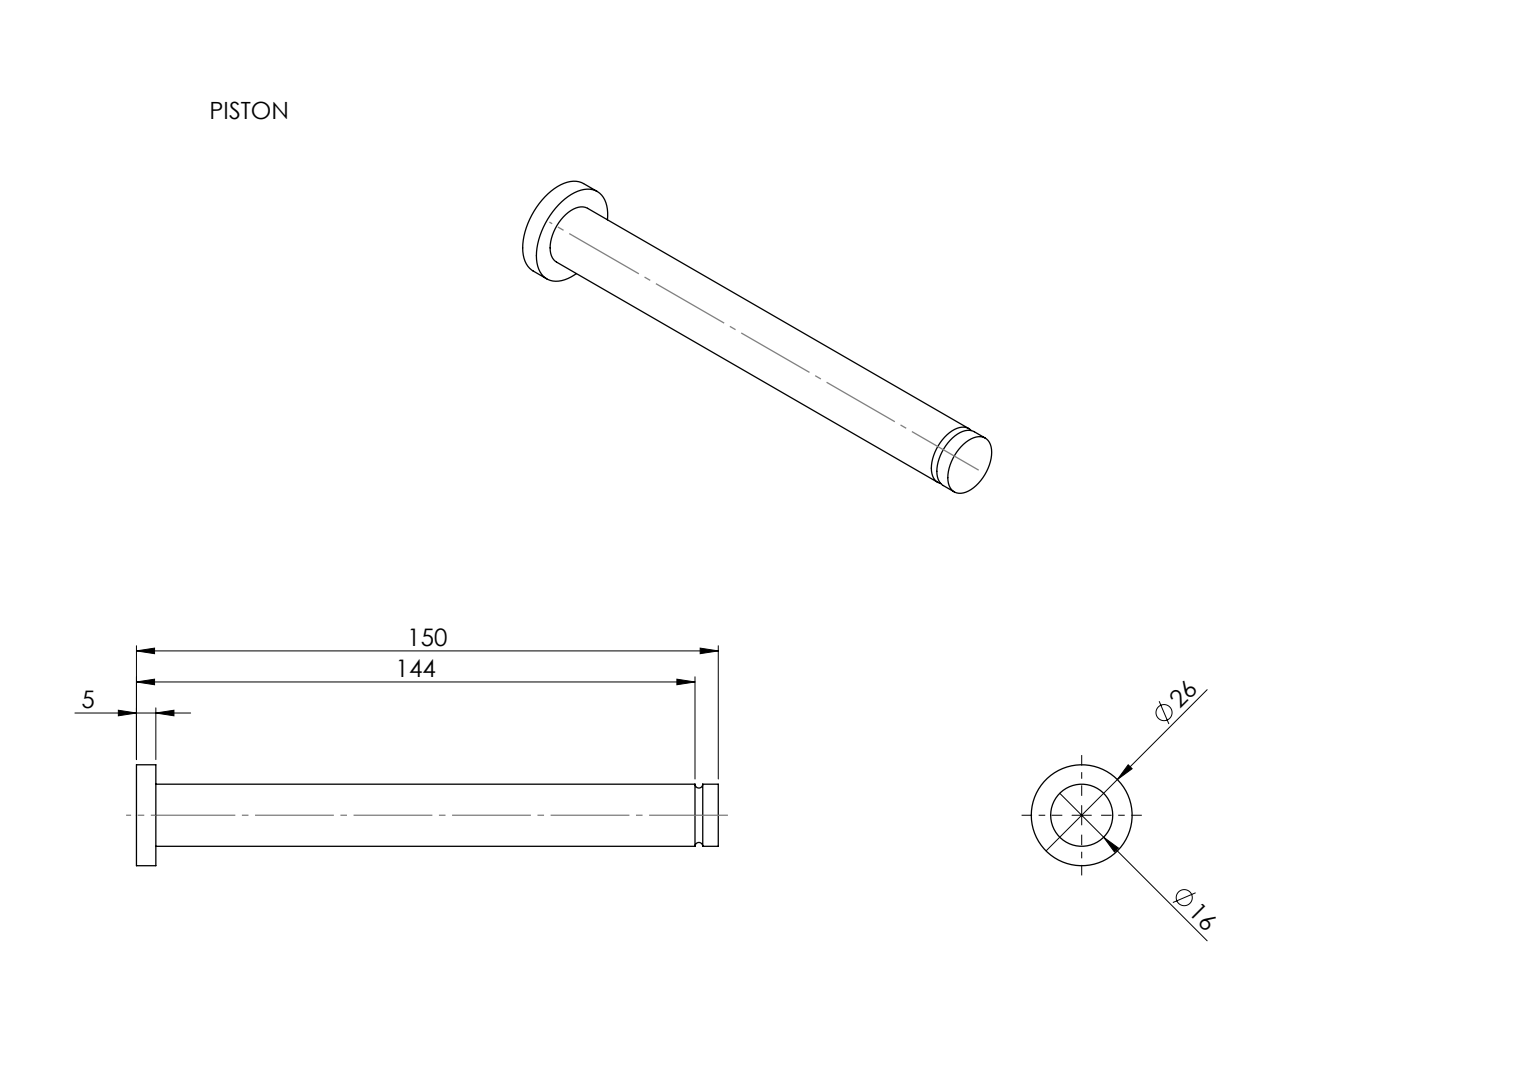
ISO-10303-21;
HEADER;
FILE_DESCRIPTION (('STEP AP214'),
    '1' );
FILE_NAME ('piston.step',
    '2026-10-08T13:22:57',
    ( '' ),
    ( '' ),
    'SwSTEP 2.0',
    'SolidWorks 2026',
    '' );
FILE_SCHEMA (( 'AUTOMOTIVE_DESIGN' ));
ENDSEC;

DATA;
#18=AXIS2_PLACEMENT_3D ( 'NONE', #9607, #4018, #5606 ) ;
#52=CIRCLE ( 'NONE', #2688, 13.00000000000000000 ) ;
#70=DIRECTION ( 'NONE',  ( 0.000000000000000000, 0.000000000000000000, 1.000000000000000000 ) ) ;
#115=ORIENTED_EDGE ( 'NONE', *, *, #1311, .F. ) ;
#116=STYLED_ITEM ( 'NONE', ( #9052 ), #3700 ) ;
#154=ORIENTED_EDGE ( 'NONE', *, *, #7460, .T. ) ;
#166=VERTEX_POINT ( 'NONE', #3235 ) ;
#178=ADVANCED_FACE ( 'NONE', ( #1639 ), #6426, .T. ) ;
#212=DIRECTION ( 'NONE',  ( 0.000000000000000000, -1.224646799147353454E-16, 1.000000000000000000 ) ) ;
#224=LINE ( 'NONE', #5694, #1710 ) ;
#245=CARTESIAN_POINT ( 'NONE',  ( 0.000000000000000000, 0.000000000000000000, 0.000000000000000000 ) ) ;
#252=ORIENTED_EDGE ( 'NONE', *, *, #5467, .F. ) ;
#395=CARTESIAN_POINT ( 'NONE',  ( 56.99999999999997158, 0.000000000000000000, 0.000000000000000000 ) ) ;
#422=DIRECTION ( 'NONE',  ( -1.000000000000000000, -0.000000000000000000, -0.000000000000000000 ) ) ;
#457=EDGE_CURVE ( 'NONE', #4209, #166, #5446, .T. ) ;
#458=ORIENTED_EDGE ( 'NONE', *, *, #1070, .T. ) ;
#467=EDGE_LOOP ( 'NONE', ( #5213, #7257 ) ) ;
#481=DIRECTION ( 'NONE',  ( 0.000000000000000000, -1.000000000000000000, 0.000000000000000000 ) ) ;
#568=ADVANCED_BREP_SHAPE_REPRESENTATION ( '', ( #3700, #3995 ), #9548 ) ;
#570=AXIS2_PLACEMENT_3D ( 'NONE', #1238, #4444, #4391 ) ;
#580=SHAPE_REPRESENTATION_RELATIONSHIP ( 'NONE' , 'NONE' ,  #8907, #568 ) ;
#635=COLOUR_RGB ( '', 0.09019608, 0.27058824, 0.51372549) ;
#653=DIRECTION ( 'NONE',  ( -1.000000000000000000, 0.000000000000000000, -0.000000000000000000 ) ) ;
#661=DIRECTION ( 'NONE',  ( -1.000000000000000000, -0.000000000000000000, -0.000000000000000000 ) ) ;
#689=AXIS2_PLACEMENT_3D ( 'NONE', #1610, #4761, #212 ) ;
#704=CYLINDRICAL_SURFACE ( 'NONE', #8270, 8.000000000000000000 ) ;
#754=DIRECTION ( 'NONE',  ( -1.000000000000000000, -0.000000000000000000, -0.000000000000000000 ) ) ;
#784=ORIENTED_EDGE ( 'NONE', *, *, #8505, .T. ) ;
#788=CARTESIAN_POINT ( 'NONE',  ( 56.99999999999997158, 0.000000000000000000, 8.000000000000000000 ) ) ;
#813=UNCERTAINTY_MEASURE_WITH_UNIT (LENGTH_MEASURE( 1.000000000000000082E-05 ), #5110, 'distance_accuracy_value', 'NONE');
#844=FACE_OUTER_BOUND ( 'NONE', #5304, .T. ) ;
#928=VERTEX_POINT ( 'NONE', #4806 ) ;
#948=DIRECTION ( 'NONE',  ( -1.000000000000000000, -0.000000000000000000, -0.000000000000000000 ) ) ;
#980=ORIENTED_EDGE ( 'NONE', *, *, #1070, .F. ) ;
#1002=CARTESIAN_POINT ( 'NONE',  ( 56.99999999999997158, 0.000000000000000000, 0.000000000000000000 ) ) ;
#1027=TOROIDAL_SURFACE ( 'NONE', #1374, 8.000000000000000000, 1.000000000000000888 ) ;
#1037=ADVANCED_FACE ( 'NONE', ( #8531 ), #4657, .T. ) ;
#1059=CARTESIAN_POINT ( 'NONE',  ( 56.99999999999997158, 0.000000000000000000, 0.000000000000000000 ) ) ;
#1068=CIRCLE ( 'NONE', #6816, 8.000000000000000000 ) ;
#1070=EDGE_CURVE ( 'NONE', #9896, #4112, #1160, .T. ) ;
#1101=SURFACE_STYLE_USAGE ( .BOTH. , #1873 ) ;
#1108=CARTESIAN_POINT ( 'NONE',  ( -83.00000000000001421, 0.000000000000000000, 0.000000000000000000 ) ) ;
#1160=CIRCLE ( 'NONE', #5118, 1.000000000000000888 ) ;
#1238=CARTESIAN_POINT ( 'NONE',  ( -88.00000000000002842, 0.000000000000000000, 0.000000000000000000 ) ) ;
#1311=EDGE_CURVE ( 'NONE', #9896, #7728, #8253, .T. ) ;
#1317=DIRECTION ( 'NONE',  ( 0.000000000000000000, 0.000000000000000000, 1.000000000000000000 ) ) ;
#1370=CARTESIAN_POINT ( 'NONE',  ( -88.00000000000002842, 0.000000000000000000, 0.000000000000000000 ) ) ;
#1374=AXIS2_PLACEMENT_3D ( 'NONE', #1059, #5794, #8174 ) ;
#1408=CARTESIAN_POINT ( 'NONE',  ( -88.00000000000002842, 0.000000000000000000, 8.000000000000000000 ) ) ;
#1416=DIRECTION ( 'NONE',  ( -1.000000000000000000, -0.000000000000000000, -0.000000000000000000 ) ) ;
#1423=EDGE_LOOP ( 'NONE', ( #9348, #2777, #5681, #2103 ) ) ;
#1425=DIRECTION ( 'NONE',  ( 0.000000000000000000, 0.000000000000000000, 1.000000000000000000 ) ) ;
#1482=CARTESIAN_POINT ( 'NONE',  ( 56.99999999999997158, 0.000000000000000000, 6.999999999999999112 ) ) ;
#1486=CARTESIAN_POINT ( 'NONE',  ( 57.99999999999997158, 0.000000000000000000, 8.000000000000000000 ) ) ;
#1526=AXIS2_PLACEMENT_3D ( 'NONE', #4077, #8682, #4034 ) ;
#1553=ORIENTED_EDGE ( 'NONE', *, *, #2011, .T. ) ;
#1569=DIRECTION ( 'NONE',  ( 0.000000000000000000, 0.000000000000000000, -1.000000000000000000 ) ) ;
#1589=DIRECTION ( 'NONE',  ( -1.000000000000000000, -0.000000000000000000, -0.000000000000000000 ) ) ;
#1610=CARTESIAN_POINT ( 'NONE',  ( 56.99999999999997158, 9.797174393178825657E-16, -8.000000000000000000 ) ) ;
#1639=FACE_OUTER_BOUND ( 'NONE', #6518, .T. ) ;
#1662=AXIS2_PLACEMENT_3D ( 'NONE', #3535, #4306, #3624 ) ;
#1692=VERTEX_POINT ( 'NONE', #7477 ) ;
#1705=VERTEX_POINT ( 'NONE', #2871 ) ;
#1710=VECTOR ( 'NONE', #8816, 1000.000000000000000 ) ;
#1810=VERTEX_POINT ( 'NONE', #1486 ) ;
#1822=DIRECTION ( 'NONE',  ( -1.000000000000000000, -0.000000000000000000, -0.000000000000000000 ) ) ;
#1833=CIRCLE ( 'NONE', #2488, 8.000000000000000000 ) ;
#1864=DIRECTION ( 'NONE',  ( -1.000000000000000000, -0.000000000000000000, -0.000000000000000000 ) ) ;
#1873=SURFACE_SIDE_STYLE ('',( #8961 ) ) ;
#1913=SURFACE_SIDE_STYLE ('',( #7386 ) ) ;
#1914=CARTESIAN_POINT ( 'NONE',  ( 55.99999999999996447, 0.000000000000000000, 0.000000000000000000 ) ) ;
#1984=DIRECTION ( 'NONE',  ( -1.000000000000000000, -0.000000000000000000, -0.000000000000000000 ) ) ;
#1985=CIRCLE ( 'NONE', #2326, 8.000000000000000000 ) ;
#2011=EDGE_CURVE ( 'NONE', #1692, #2905, #7742, .T. ) ;
#2027=CARTESIAN_POINT ( 'NONE',  ( 56.99999999999997158, 0.000000000000000000, 8.000000000000000000 ) ) ;
#2033=DIRECTION ( 'NONE',  ( 0.000000000000000000, 0.000000000000000000, 1.000000000000000000 ) ) ;
#2054=ORIENTED_EDGE ( 'NONE', *, *, #3567, .F. ) ;
#2061=EDGE_LOOP ( 'NONE', ( #252, #784, #3897, #9819 ) ) ;
#2103=ORIENTED_EDGE ( 'NONE', *, *, #6989, .F. ) ;
#2126=EDGE_CURVE ( 'NONE', #9861, #928, #5621, .T. ) ;
#2163=CIRCLE ( 'NONE', #3319, 6.999999999999999112 ) ;
#2196=ORIENTED_EDGE ( 'NONE', *, *, #2684, .F. ) ;
#2248=DIRECTION ( 'NONE',  ( -0.000000000000000000, 0.000000000000000000, 1.000000000000000000 ) ) ;
#2269=ORIENTED_EDGE ( 'NONE', *, *, #5485, .T. ) ;
#2326=AXIS2_PLACEMENT_3D ( 'NONE', #4570, #9220, #7774 ) ;
#2380=AXIS2_PLACEMENT_3D ( 'NONE', #788, #4715, #1569 ) ;
#2390=CARTESIAN_POINT ( 'NONE',  ( -83.00000000000001421, 9.797174393178825657E-16, -8.000000000000000000 ) ) ;
#2395=FACE_OUTER_BOUND ( 'NONE', #1423, .T. ) ;
#2424=CARTESIAN_POINT ( 'NONE',  ( -83.00000000000001421, 0.000000000000000000, 13.00000000000000000 ) ) ;
#2488=AXIS2_PLACEMENT_3D ( 'NONE', #8057, #7287, #3931 ) ;
#2535=EDGE_CURVE ( 'NONE', #2905, #166, #5283, .T. ) ;
#2550=DIRECTION ( 'NONE',  ( 0.000000000000000000, 0.000000000000000000, 1.000000000000000000 ) ) ;
#2591=DIRECTION ( 'NONE',  ( 0.000000000000000000, 0.000000000000000000, 1.000000000000000000 ) ) ;
#2597=DIRECTION ( 'NONE',  ( 0.000000000000000000, 0.000000000000000000, 1.000000000000000000 ) ) ;
#2611=PRODUCT_DEFINITION_FORMATION_WITH_SPECIFIED_SOURCE ( 'ANY', '', #6639, .NOT_KNOWN. ) ;
#2682=CIRCLE ( 'NONE', #6305, 8.000000000000000000 ) ;
#2684=EDGE_CURVE ( 'NONE', #1705, #6462, #3540, .T. ) ;
#2688=AXIS2_PLACEMENT_3D ( 'NONE', #7784, #754, #70 ) ;
#2749=MECHANICAL_DESIGN_GEOMETRIC_PRESENTATION_REPRESENTATION('',(#116),#3578);
#2768=VERTEX_POINT ( 'NONE', #3014 ) ;
#2777=ORIENTED_EDGE ( 'NONE', *, *, #6679, .T. ) ;
#2800=ORIENTED_EDGE ( 'NONE', *, *, #4948, .F. ) ;
#2851=FACE_OUTER_BOUND ( 'NONE', #8992, .T. ) ;
#2860=PLANE ( 'NONE',  #9099 ) ;
#2869=ADVANCED_FACE ( 'NONE', ( #2395 ), #704, .T. ) ;
#2871=CARTESIAN_POINT ( 'NONE',  ( 55.99999999999996447, 0.000000000000000000, 8.000000000000000000 ) ) ;
#2905=VERTEX_POINT ( 'NONE', #9384 ) ;
#2973=ORIENTED_EDGE ( 'NONE', *, *, #8348, .T. ) ;
#2981=AXIS2_PLACEMENT_3D ( 'NONE', #7760, #6860, #10083 ) ;
#2991=ORIENTED_EDGE ( 'NONE', *, *, #457, .F. ) ;
#3014=CARTESIAN_POINT ( 'NONE',  ( 55.99999999999996447, 9.797174393178825657E-16, -8.000000000000000000 ) ) ;
#3018=CIRCLE ( 'NONE', #6628, 13.00000000000000000 ) ;
#3050=PLANE ( 'NONE',  #2981 ) ;
#3089=COLOUR_RGB ( '', 0.09019608, 0.27058824, 0.51372549) ;
#3099=DIRECTION ( 'NONE',  ( 0.000000000000000000, 0.000000000000000000, 1.000000000000000000 ) ) ;
#3101=DIRECTION ( 'NONE',  ( -1.000000000000000000, -0.000000000000000000, -0.000000000000000000 ) ) ;
#3146=CIRCLE ( 'NONE', #5278, 8.000000000000000000 ) ;
#3183=EDGE_LOOP ( 'NONE', ( #115, #458, #8887, #6583 ) ) ;
#3210=AXIS2_PLACEMENT_3D ( 'NONE', #6299, #1416, #8541 ) ;
#3231=ORIENTED_EDGE ( 'NONE', *, *, #2126, .T. ) ;
#3235=CARTESIAN_POINT ( 'NONE',  ( -88.00000000000002842, 0.000000000000000000, 13.00000000000000000 ) ) ;
#3237=DIRECTION ( 'NONE',  ( -1.000000000000000000, -0.000000000000000000, -0.000000000000000000 ) ) ;
#3318=AXIS2_PLACEMENT_3D ( 'NONE', #1370, #9952, #2033 ) ;
#3319=AXIS2_PLACEMENT_3D ( 'NONE', #395, #8295, #5806 ) ;
#3353=ORIENTED_EDGE ( 'NONE', *, *, #1311, .T. ) ;
#3377=DIRECTION ( 'NONE',  ( -1.000000000000000000, -0.000000000000000000, -0.000000000000000000 ) ) ;
#3429=ORIENTED_EDGE ( 'NONE', *, *, #6679, .F. ) ;
#3494=PRODUCT_DEFINITION_CONTEXT ( 'detailed design', #4873, 'design' ) ;
#3535=CARTESIAN_POINT ( 'NONE',  ( -83.00000000000001421, 0.000000000000000000, 13.00000000000000000 ) ) ;
#3540=LINE ( 'NONE', #8290, #6746 ) ;
#3567=EDGE_CURVE ( 'NONE', #1705, #2768, #8869, .T. ) ;
#3578=( GEOMETRIC_REPRESENTATION_CONTEXT ( 3 ) GLOBAL_UNCERTAINTY_ASSIGNED_CONTEXT ( ( #813 ) ) GLOBAL_UNIT_ASSIGNED_CONTEXT ( ( #5110, #4336, #5926 ) ) REPRESENTATION_CONTEXT ( 'NONE', 'WORKASPACE' ) );
#3623=AXIS2_PLACEMENT_3D ( 'NONE', #3929, #7855, #3099 ) ;
#3624=DIRECTION ( 'NONE',  ( 0.000000000000000000, 0.000000000000000000, -1.000000000000000000 ) ) ;
#3660=CLOSED_SHELL ( 'NONE', ( #4316, #9400, #6703, #5314, #178, #6131, #7297, #8672, #8192, #2869, #5187, #1037, #9746 ) ) ;
#3669=EDGE_CURVE ( 'NONE', #2768, #9103, #8950, .T. ) ;
#3694=DIRECTION ( 'NONE',  ( -1.000000000000000000, -0.000000000000000000, -0.000000000000000000 ) ) ;
#3700=MANIFOLD_SOLID_BREP ( 'Revolve1', #3660 ) ;
#3706=ORIENTED_EDGE ( 'NONE', *, *, #2535, .F. ) ;
#3708=ORIENTED_EDGE ( 'NONE', *, *, #9778, .F. ) ;
#3874=ORIENTED_EDGE ( 'NONE', *, *, #10088, .T. ) ;
#3886=ORIENTED_EDGE ( 'NONE', *, *, #3567, .T. ) ;
#3897=ORIENTED_EDGE ( 'NONE', *, *, #9778, .T. ) ;
#3929=CARTESIAN_POINT ( 'NONE',  ( -88.00000000000002842, 0.000000000000000000, 0.000000000000000000 ) ) ;
#3931=DIRECTION ( 'NONE',  ( 0.000000000000000000, 0.000000000000000000, 1.000000000000000000 ) ) ;
#3958=ORIENTED_EDGE ( 'NONE', *, *, #5485, .F. ) ;
#3960=VECTOR ( 'NONE', #9493, 1000.000000000000000 ) ;
#3995=AXIS2_PLACEMENT_3D ( 'NONE', #245, #8930, #7419 ) ;
#3999=CYLINDRICAL_SURFACE ( 'NONE', #4635, 13.00000000000000000 ) ;
#4018=DIRECTION ( 'NONE',  ( -1.000000000000000000, -0.000000000000000000, -0.000000000000000000 ) ) ;
#4034=DIRECTION ( 'NONE',  ( 0.000000000000000000, 0.000000000000000000, 1.000000000000000000 ) ) ;
#4077=CARTESIAN_POINT ( 'NONE',  ( 56.99999999999997158, 0.000000000000000000, 0.000000000000000000 ) ) ;
#4110=DIRECTION ( 'NONE',  ( 0.000000000000000000, 0.000000000000000000, 1.000000000000000000 ) ) ;
#4112=VERTEX_POINT ( 'NONE', #6491 ) ;
#4209=VERTEX_POINT ( 'NONE', #2424 ) ;
#4233=FILL_AREA_STYLE ('',( #8159 ) ) ;
#4285=SURFACE_STYLE_USAGE ( .BOTH. , #1913 ) ;
#4306=DIRECTION ( 'NONE',  ( 1.000000000000000000, 0.000000000000000000, 0.000000000000000000 ) ) ;
#4316=ADVANCED_FACE ( 'NONE', ( #4802 ), #8796, .F. ) ;
#4336=( NAMED_UNIT ( * ) PLANE_ANGLE_UNIT ( ) SI_UNIT ( $, .RADIAN. ) );
#4360=EDGE_LOOP ( 'NONE', ( #3231, #5060, #5358, #3708 ) ) ;
#4391=DIRECTION ( 'NONE',  ( 0.000000000000000000, 0.000000000000000000, 1.000000000000000000 ) ) ;
#4444=DIRECTION ( 'NONE',  ( -1.000000000000000000, -0.000000000000000000, -0.000000000000000000 ) ) ;
#4570=CARTESIAN_POINT ( 'NONE',  ( 61.99999999999997158, 0.000000000000000000, 0.000000000000000000 ) ) ;
#4635=AXIS2_PLACEMENT_3D ( 'NONE', #9486, #948, #2591 ) ;
#4637=CARTESIAN_POINT ( 'NONE',  ( -88.00000000000002842, 1.592040838891559095E-15, -13.00000000000000000 ) ) ;
#4657=CYLINDRICAL_SURFACE ( 'NONE', #3623, 8.000000000000000000 ) ;
#4715=DIRECTION ( 'NONE',  ( 0.000000000000000000, -1.000000000000000000, 0.000000000000000000 ) ) ;
#4761=DIRECTION ( 'NONE',  ( -0.000000000000000000, 1.000000000000000000, 1.224646799147353207E-16 ) ) ;
#4800=AXIS2_PLACEMENT_3D ( 'NONE', #8667, #1589, #7108 ) ;
#4802=FACE_OUTER_BOUND ( 'NONE', #9503, .T. ) ;
#4806=CARTESIAN_POINT ( 'NONE',  ( 61.99999999999997158, 9.797174393178825657E-16, -8.000000000000000000 ) ) ;
#4873=APPLICATION_CONTEXT ( 'automotive_design' ) ;
#4891=DIRECTION ( 'NONE',  ( 0.000000000000000000, 0.000000000000000000, 1.000000000000000000 ) ) ;
#4948=EDGE_CURVE ( 'NONE', #166, #2905, #52, .T. ) ;
#4966=ORIENTED_EDGE ( 'NONE', *, *, #9912, .T. ) ;
#5012=ORIENTED_EDGE ( 'NONE', *, *, #7460, .F. ) ;
#5013=CARTESIAN_POINT ( 'NONE',  ( -88.00000000000002842, 9.797174393178825657E-16, -8.000000000000000000 ) ) ;
#5060=ORIENTED_EDGE ( 'NONE', *, *, #5467, .T. ) ;
#5062=DIRECTION ( 'NONE',  ( 0.000000000000000000, 0.000000000000000000, 1.000000000000000000 ) ) ;
#5089=FACE_OUTER_BOUND ( 'NONE', #467, .T. ) ;
#5110=( LENGTH_UNIT ( ) NAMED_UNIT ( * ) SI_UNIT ( .MILLI., .METRE. ) );
#5118=AXIS2_PLACEMENT_3D ( 'NONE', #9417, #7073, #9316 ) ;
#5120=( NAMED_UNIT ( * ) PLANE_ANGLE_UNIT ( ) SI_UNIT ( $, .RADIAN. ) );
#5131=VECTOR ( 'NONE', #3101, 1000.000000000000000 ) ;
#5177=PRODUCT_DEFINITION_SHAPE ( 'NONE', 'NONE',  #9415 ) ;
#5187=ADVANCED_FACE ( 'NONE', ( #9337 ), #1027, .F. ) ;
#5213=ORIENTED_EDGE ( 'NONE', *, *, #4948, .T. ) ;
#5278=AXIS2_PLACEMENT_3D ( 'NONE', #5584, #9533, #7243 ) ;
#5283=CIRCLE ( 'NONE', #3318, 13.00000000000000000 ) ;
#5304=EDGE_LOOP ( 'NONE', ( #7513, #2269, #8105, #3706 ) ) ;
#5314=ADVANCED_FACE ( 'NONE', ( #7302 ), #7146, .F. ) ;
#5328=LINE ( 'NONE', #1408, #5131 ) ;
#5330=PRESENTATION_STYLE_ASSIGNMENT (( #1101 ) ) ;
#5358=ORIENTED_EDGE ( 'NONE', *, *, #8807, .F. ) ;
#5360=ORIENTED_EDGE ( 'NONE', *, *, #7171, .F. ) ;
#5388=ORIENTED_EDGE ( 'NONE', *, *, #7171, .T. ) ;
#5408=( GEOMETRIC_REPRESENTATION_CONTEXT ( 3 ) GLOBAL_UNCERTAINTY_ASSIGNED_CONTEXT ( ( #9905 ) ) GLOBAL_UNIT_ASSIGNED_CONTEXT ( ( #5427, #5482, #7858 ) ) REPRESENTATION_CONTEXT ( 'NONE', 'WORKASPACE' ) );
#5427=( LENGTH_UNIT ( ) NAMED_UNIT ( * ) SI_UNIT ( .MILLI., .METRE. ) );
#5443=EDGE_CURVE ( 'NONE', #4112, #1810, #2682, .T. ) ;
#5446=LINE ( 'NONE', #8607, #3960 ) ;
#5467=EDGE_CURVE ( 'NONE', #928, #4112, #224, .T. ) ;
#5482=( NAMED_UNIT ( * ) PLANE_ANGLE_UNIT ( ) SI_UNIT ( $, .RADIAN. ) );
#5485=EDGE_CURVE ( 'NONE', #1692, #4209, #3018, .T. ) ;
#5584=CARTESIAN_POINT ( 'NONE',  ( 57.99999999999997158, 0.000000000000000000, 0.000000000000000000 ) ) ;
#5606=DIRECTION ( 'NONE',  ( 0.000000000000000000, 0.000000000000000000, 1.000000000000000000 ) ) ;
#5621=CIRCLE ( 'NONE', #4800, 8.000000000000000000 ) ;
#5681=ORIENTED_EDGE ( 'NONE', *, *, #2684, .T. ) ;
#5694=CARTESIAN_POINT ( 'NONE',  ( -88.00000000000002842, 9.797174393178825657E-16, -8.000000000000000000 ) ) ;
#5735=MECHANICAL_DESIGN_GEOMETRIC_PRESENTATION_REPRESENTATION('',(#7384),#5408);
#5740=DIRECTION ( 'NONE',  ( -1.000000000000000000, -0.000000000000000000, -0.000000000000000000 ) ) ;
#5779=CARTESIAN_POINT ( 'NONE',  ( -83.00000000000001421, 0.000000000000000000, 8.000000000000000000 ) ) ;
#5787=FILL_AREA_STYLE_COLOUR ( '', #635 ) ;
#5794=DIRECTION ( 'NONE',  ( -1.000000000000000000, -0.000000000000000000, -0.000000000000000000 ) ) ;
#5806=DIRECTION ( 'NONE',  ( 0.000000000000000000, 0.000000000000000000, 1.000000000000000000 ) ) ;
#5926=( NAMED_UNIT ( * ) SI_UNIT ( $, .STERADIAN. ) SOLID_ANGLE_UNIT ( ) );
#5979=DIRECTION ( 'NONE',  ( -1.000000000000000000, -0.000000000000000000, -0.000000000000000000 ) ) ;
#6034=EDGE_CURVE ( 'NONE', #1705, #7728, #6992, .T. ) ;
#6068=ORIENTED_EDGE ( 'NONE', *, *, #2126, .F. ) ;
#6131=ADVANCED_FACE ( 'NONE', ( #10193 ), #8694, .T. ) ;
#6207=ORIENTED_EDGE ( 'NONE', *, *, #6034, .T. ) ;
#6299=CARTESIAN_POINT ( 'NONE',  ( -88.00000000000002842, 0.000000000000000000, 0.000000000000000000 ) ) ;
#6305=AXIS2_PLACEMENT_3D ( 'NONE', #8023, #5740, #9688 ) ;
#6318=ORIENTED_EDGE ( 'NONE', *, *, #6034, .F. ) ;
#6426=CYLINDRICAL_SURFACE ( 'NONE', #18, 8.000000000000000000 ) ;
#6443=AXIS2_PLACEMENT_3D ( 'NONE', #8164, #422, #7392 ) ;
#6462=VERTEX_POINT ( 'NONE', #5779 ) ;
#6491=CARTESIAN_POINT ( 'NONE',  ( 57.99999999999997158, 9.797174393178825657E-16, -8.000000000000000000 ) ) ;
#6518=EDGE_LOOP ( 'NONE', ( #3886, #9205, #8618, #2196 ) ) ;
#6574=UNCERTAINTY_MEASURE_WITH_UNIT (LENGTH_MEASURE( 1.000000000000000082E-05 ), #6809, 'distance_accuracy_value', 'NONE');
#6583=ORIENTED_EDGE ( 'NONE', *, *, #8348, .F. ) ;
#6596=CARTESIAN_POINT ( 'NONE',  ( 55.99999999999996447, 0.000000000000000000, 0.000000000000000000 ) ) ;
#6628=AXIS2_PLACEMENT_3D ( 'NONE', #1108, #3377, #2550 ) ;
#6639=PRODUCT ( 'piston', 'piston', '', ( #9869 ) ) ;
#6679=EDGE_CURVE ( 'NONE', #2768, #1705, #1068, .T. ) ;
#6690=DIRECTION ( 'NONE',  ( 0.000000000000000000, 0.000000000000000000, 1.000000000000000000 ) ) ;
#6703=ADVANCED_FACE ( 'NONE', ( #8320 ), #7595, .T. ) ;
#6746=VECTOR ( 'NONE', #1984, 1000.000000000000000 ) ;
#6809=( LENGTH_UNIT ( ) NAMED_UNIT ( * ) SI_UNIT ( .MILLI., .METRE. ) );
#6816=AXIS2_PLACEMENT_3D ( 'NONE', #1914, #5979, #5062 ) ;
#6842=CARTESIAN_POINT ( 'NONE',  ( -83.00000000000001421, 0.000000000000000000, 0.000000000000000000 ) ) ;
#6860=DIRECTION ( 'NONE',  ( 1.000000000000000000, 0.000000000000000000, 0.000000000000000000 ) ) ;
#6929=EDGE_LOOP ( 'NONE', ( #6068, #8870 ) ) ;
#6989=EDGE_CURVE ( 'NONE', #9103, #6462, #8434, .T. ) ;
#6992=CIRCLE ( 'NONE', #2380, 1.000000000000000888 ) ;
#7027=FACE_OUTER_BOUND ( 'NONE', #6929, .T. ) ;
#7051=DIRECTION ( 'NONE',  ( -1.000000000000000000, -0.000000000000000000, -0.000000000000000000 ) ) ;
#7073=DIRECTION ( 'NONE',  ( -0.000000000000000000, 1.000000000000000000, 1.224646799147353207E-16 ) ) ;
#7108=DIRECTION ( 'NONE',  ( 0.000000000000000000, 0.000000000000000000, 1.000000000000000000 ) ) ;
#7146=TOROIDAL_SURFACE ( 'NONE', #7474, 8.000000000000000000, 1.000000000000000888 ) ;
#7171=EDGE_CURVE ( 'NONE', #7728, #9896, #2163, .T. ) ;
#7243=DIRECTION ( 'NONE',  ( 0.000000000000000000, 0.000000000000000000, 1.000000000000000000 ) ) ;
#7257=ORIENTED_EDGE ( 'NONE', *, *, #2535, .T. ) ;
#7279=CIRCLE ( 'NONE', #9600, 13.00000000000000000 ) ;
#7287=DIRECTION ( 'NONE',  ( -1.000000000000000000, -0.000000000000000000, -0.000000000000000000 ) ) ;
#7297=ADVANCED_FACE ( 'NONE', ( #5089 ), #2860, .T. ) ;
#7302=FACE_OUTER_BOUND ( 'NONE', #3183, .T. ) ;
#7384=STYLED_ITEM ( 'NONE', ( #5330 ), #568 ) ;
#7386=SURFACE_STYLE_FILL_AREA ( #4233 ) ;
#7392=DIRECTION ( 'NONE',  ( 0.000000000000000000, 0.000000000000000000, 1.000000000000000000 ) ) ;
#7419=DIRECTION ( 'NONE',  ( 1.000000000000000000, 0.000000000000000000, 0.000000000000000000 ) ) ;
#7460=EDGE_CURVE ( 'NONE', #4209, #1692, #7279, .T. ) ;
#7474=AXIS2_PLACEMENT_3D ( 'NONE', #1002, #1822, #2597 ) ;
#7477=CARTESIAN_POINT ( 'NONE',  ( -83.00000000000001421, 1.592040838891559095E-15, -13.00000000000000000 ) ) ;
#7513=ORIENTED_EDGE ( 'NONE', *, *, #2011, .F. ) ;
#7595=CYLINDRICAL_SURFACE ( 'NONE', #570, 8.000000000000000000 ) ;
#7611=CIRCLE ( 'NONE', #689, 1.000000000000000888 ) ;
#7714=VECTOR ( 'NONE', #1864, 1000.000000000000000 ) ;
#7728=VERTEX_POINT ( 'NONE', #1482 ) ;
#7742=LINE ( 'NONE', #4637, #8093 ) ;
#7760=CARTESIAN_POINT ( 'NONE',  ( 61.99999999999997158, 0.000000000000000000, 8.000000000000000000 ) ) ;
#7774=DIRECTION ( 'NONE',  ( 0.000000000000000000, 0.000000000000000000, 1.000000000000000000 ) ) ;
#7784=CARTESIAN_POINT ( 'NONE',  ( -88.00000000000002842, 0.000000000000000000, 0.000000000000000000 ) ) ;
#7855=DIRECTION ( 'NONE',  ( -1.000000000000000000, -0.000000000000000000, -0.000000000000000000 ) ) ;
#7858=( NAMED_UNIT ( * ) SI_UNIT ( $, .STERADIAN. ) SOLID_ANGLE_UNIT ( ) );
#7924=AXIS2_PLACEMENT_3D ( 'NONE', #2027, #481, #10098 ) ;
#7974=ORIENTED_EDGE ( 'NONE', *, *, #6989, .T. ) ;
#8020=EDGE_LOOP ( 'NONE', ( #5360, #2973, #9155, #980 ) ) ;
#8023=CARTESIAN_POINT ( 'NONE',  ( 57.99999999999997158, 0.000000000000000000, 0.000000000000000000 ) ) ;
#8057=CARTESIAN_POINT ( 'NONE',  ( -83.00000000000001421, 0.000000000000000000, 0.000000000000000000 ) ) ;
#8093=VECTOR ( 'NONE', #661, 1000.000000000000000 ) ;
#8105=ORIENTED_EDGE ( 'NONE', *, *, #457, .T. ) ;
#8159=FILL_AREA_STYLE_COLOUR ( '', #3089 ) ;
#8164=CARTESIAN_POINT ( 'NONE',  ( 56.99999999999997158, 0.000000000000000000, 0.000000000000000000 ) ) ;
#8174=DIRECTION ( 'NONE',  ( 0.000000000000000000, 0.000000000000000000, 1.000000000000000000 ) ) ;
#8192=ADVANCED_FACE ( 'NONE', ( #8384, #2851 ), #9892, .T. ) ;
#8200=AXIS2_PLACEMENT_3D ( 'NONE', #6596, #9002, #6690 ) ;
#8253=CIRCLE ( 'NONE', #9254, 6.999999999999999112 ) ;
#8270=AXIS2_PLACEMENT_3D ( 'NONE', #9490, #10047, #1425 ) ;
#8273=( NAMED_UNIT ( * ) SI_UNIT ( $, .STERADIAN. ) SOLID_ANGLE_UNIT ( ) );
#8290=CARTESIAN_POINT ( 'NONE',  ( -88.00000000000002842, 0.000000000000000000, 8.000000000000000000 ) ) ;
#8295=DIRECTION ( 'NONE',  ( -1.000000000000000000, -0.000000000000000000, -0.000000000000000000 ) ) ;
#8318=ORIENTED_EDGE ( 'NONE', *, *, #10088, .F. ) ;
#8320=FACE_OUTER_BOUND ( 'NONE', #4360, .T. ) ;
#8348=EDGE_CURVE ( 'NONE', #7728, #1810, #8929, .T. ) ;
#8375=FILL_AREA_STYLE ('',( #5787 ) ) ;
#8384=FACE_BOUND ( 'NONE', #8850, .T. ) ;
#8402=EDGE_LOOP ( 'NONE', ( #154, #1553, #2800, #2991 ) ) ;
#8405=EDGE_LOOP ( 'NONE', ( #3874, #3353, #6318, #3429 ) ) ;
#8434=CIRCLE ( 'NONE', #9273, 8.000000000000000000 ) ;
#8436=TOROIDAL_SURFACE ( 'NONE', #6443, 8.000000000000000000, 1.000000000000000888 ) ;
#8505=EDGE_CURVE ( 'NONE', #928, #9861, #1985, .T. ) ;
#8531=FACE_OUTER_BOUND ( 'NONE', #2061, .T. ) ;
#8541=DIRECTION ( 'NONE',  ( 0.000000000000000000, 0.000000000000000000, 1.000000000000000000 ) ) ;
#8607=CARTESIAN_POINT ( 'NONE',  ( -88.00000000000002842, 0.000000000000000000, 13.00000000000000000 ) ) ;
#8618=ORIENTED_EDGE ( 'NONE', *, *, #9912, .F. ) ;
#8667=CARTESIAN_POINT ( 'NONE',  ( 61.99999999999997158, 0.000000000000000000, 0.000000000000000000 ) ) ;
#8672=ADVANCED_FACE ( 'NONE', ( #844 ), #3999, .T. ) ;
#8682=DIRECTION ( 'NONE',  ( -1.000000000000000000, -0.000000000000000000, -0.000000000000000000 ) ) ;
#8694=CYLINDRICAL_SURFACE ( 'NONE', #3210, 13.00000000000000000 ) ;
#8770=APPLICATION_CONTEXT ( 'automotive_design' ) ;
#8795=CARTESIAN_POINT ( 'NONE',  ( 56.99999999999997158, 8.572527594031471218E-16, -6.999999999999999112 ) ) ;
#8796=TOROIDAL_SURFACE ( 'NONE', #1526, 8.000000000000000000, 1.000000000000000888 ) ;
#8807=EDGE_CURVE ( 'NONE', #1810, #4112, #3146, .T. ) ;
#8816=DIRECTION ( 'NONE',  ( -1.000000000000000000, -0.000000000000000000, -0.000000000000000000 ) ) ;
#8850=EDGE_LOOP ( 'NONE', ( #4966, #7974 ) ) ;
#8869=CIRCLE ( 'NONE', #8200, 8.000000000000000000 ) ;
#8870=ORIENTED_EDGE ( 'NONE', *, *, #8505, .F. ) ;
#8887=ORIENTED_EDGE ( 'NONE', *, *, #5443, .T. ) ;
#8907=SHAPE_REPRESENTATION ( 'piston', ( #3995 ), #9548 ) ;
#8929=CIRCLE ( 'NONE', #7924, 1.000000000000000888 ) ;
#8930=DIRECTION ( 'NONE',  ( 0.000000000000000000, 0.000000000000000000, 1.000000000000000000 ) ) ;
#8950=LINE ( 'NONE', #5013, #7714 ) ;
#8959=FACE_OUTER_BOUND ( 'NONE', #8405, .T. ) ;
#8961=SURFACE_STYLE_FILL_AREA ( #8375 ) ;
#8992=EDGE_LOOP ( 'NONE', ( #5012, #3958 ) ) ;
#9002=DIRECTION ( 'NONE',  ( -1.000000000000000000, -0.000000000000000000, -0.000000000000000000 ) ) ;
#9052=PRESENTATION_STYLE_ASSIGNMENT (( #4285 ) ) ;
#9099=AXIS2_PLACEMENT_3D ( 'NONE', #9289, #653, #2248 ) ;
#9103=VERTEX_POINT ( 'NONE', #2390 ) ;
#9155=ORIENTED_EDGE ( 'NONE', *, *, #8807, .T. ) ;
#9205=ORIENTED_EDGE ( 'NONE', *, *, #3669, .T. ) ;
#9220=DIRECTION ( 'NONE',  ( -1.000000000000000000, -0.000000000000000000, -0.000000000000000000 ) ) ;
#9254=AXIS2_PLACEMENT_3D ( 'NONE', #9597, #7051, #4110 ) ;
#9273=AXIS2_PLACEMENT_3D ( 'NONE', #6842, #3237, #4891 ) ;
#9289=CARTESIAN_POINT ( 'NONE',  ( -88.00000000000002842, 0.000000000000000000, 0.000000000000000000 ) ) ;
#9316=DIRECTION ( 'NONE',  ( 0.000000000000000000, -1.224646799147353454E-16, 1.000000000000000000 ) ) ;
#9337=FACE_OUTER_BOUND ( 'NONE', #8020, .T. ) ;
#9348=ORIENTED_EDGE ( 'NONE', *, *, #3669, .F. ) ;
#9384=CARTESIAN_POINT ( 'NONE',  ( -88.00000000000002842, 1.592040838891559095E-15, -13.00000000000000000 ) ) ;
#9400=ADVANCED_FACE ( 'NONE', ( #8959 ), #8436, .F. ) ;
#9415=PRODUCT_DEFINITION ( 'UNKNOWN', '', #2611, #3494 ) ;
#9417=CARTESIAN_POINT ( 'NONE',  ( 56.99999999999997158, 9.797174393178825657E-16, -8.000000000000000000 ) ) ;
#9419=CARTESIAN_POINT ( 'NONE',  ( 61.99999999999997158, 0.000000000000000000, 8.000000000000000000 ) ) ;
#9486=CARTESIAN_POINT ( 'NONE',  ( -88.00000000000002842, 0.000000000000000000, 0.000000000000000000 ) ) ;
#9490=CARTESIAN_POINT ( 'NONE',  ( -88.00000000000002842, 0.000000000000000000, 0.000000000000000000 ) ) ;
#9493=DIRECTION ( 'NONE',  ( -1.000000000000000000, -0.000000000000000000, -0.000000000000000000 ) ) ;
#9503=EDGE_LOOP ( 'NONE', ( #6207, #5388, #8318, #2054 ) ) ;
#9533=DIRECTION ( 'NONE',  ( -1.000000000000000000, -0.000000000000000000, -0.000000000000000000 ) ) ;
#9548=( GEOMETRIC_REPRESENTATION_CONTEXT ( 3 ) GLOBAL_UNCERTAINTY_ASSIGNED_CONTEXT ( ( #6574 ) ) GLOBAL_UNIT_ASSIGNED_CONTEXT ( ( #6809, #5120, #8273 ) ) REPRESENTATION_CONTEXT ( 'NONE', 'WORKASPACE' ) );
#9597=CARTESIAN_POINT ( 'NONE',  ( 56.99999999999997158, 0.000000000000000000, 0.000000000000000000 ) ) ;
#9600=AXIS2_PLACEMENT_3D ( 'NONE', #10002, #3694, #1317 ) ;
#9607=CARTESIAN_POINT ( 'NONE',  ( -88.00000000000002842, 0.000000000000000000, 0.000000000000000000 ) ) ;
#9688=DIRECTION ( 'NONE',  ( 0.000000000000000000, 0.000000000000000000, 1.000000000000000000 ) ) ;
#9746=ADVANCED_FACE ( 'NONE', ( #7027 ), #3050, .T. ) ;
#9778=EDGE_CURVE ( 'NONE', #9861, #1810, #5328, .T. ) ;
#9819=ORIENTED_EDGE ( 'NONE', *, *, #5443, .F. ) ;
#9861=VERTEX_POINT ( 'NONE', #9419 ) ;
#9869=PRODUCT_CONTEXT ( 'NONE', #8770, 'mechanical' ) ;
#9892=PLANE ( 'NONE',  #1662 ) ;
#9896=VERTEX_POINT ( 'NONE', #8795 ) ;
#9905=UNCERTAINTY_MEASURE_WITH_UNIT (LENGTH_MEASURE( 1.000000000000000082E-05 ), #5427, 'distance_accuracy_value', 'NONE');
#9912=EDGE_CURVE ( 'NONE', #6462, #9103, #1833, .T. ) ;
#9952=DIRECTION ( 'NONE',  ( -1.000000000000000000, -0.000000000000000000, -0.000000000000000000 ) ) ;
#9972=SHAPE_DEFINITION_REPRESENTATION ( #5177, #8907 ) ;
#10002=CARTESIAN_POINT ( 'NONE',  ( -83.00000000000001421, 0.000000000000000000, 0.000000000000000000 ) ) ;
#10047=DIRECTION ( 'NONE',  ( -1.000000000000000000, -0.000000000000000000, -0.000000000000000000 ) ) ;
#10083=DIRECTION ( 'NONE',  ( 0.000000000000000000, 0.000000000000000000, -1.000000000000000000 ) ) ;
#10088=EDGE_CURVE ( 'NONE', #2768, #9896, #7611, .T. ) ;
#10098=DIRECTION ( 'NONE',  ( 0.000000000000000000, 0.000000000000000000, -1.000000000000000000 ) ) ;
#10193=FACE_OUTER_BOUND ( 'NONE', #8402, .T. ) ;
ENDSEC;
END-ISO-10303-21;
